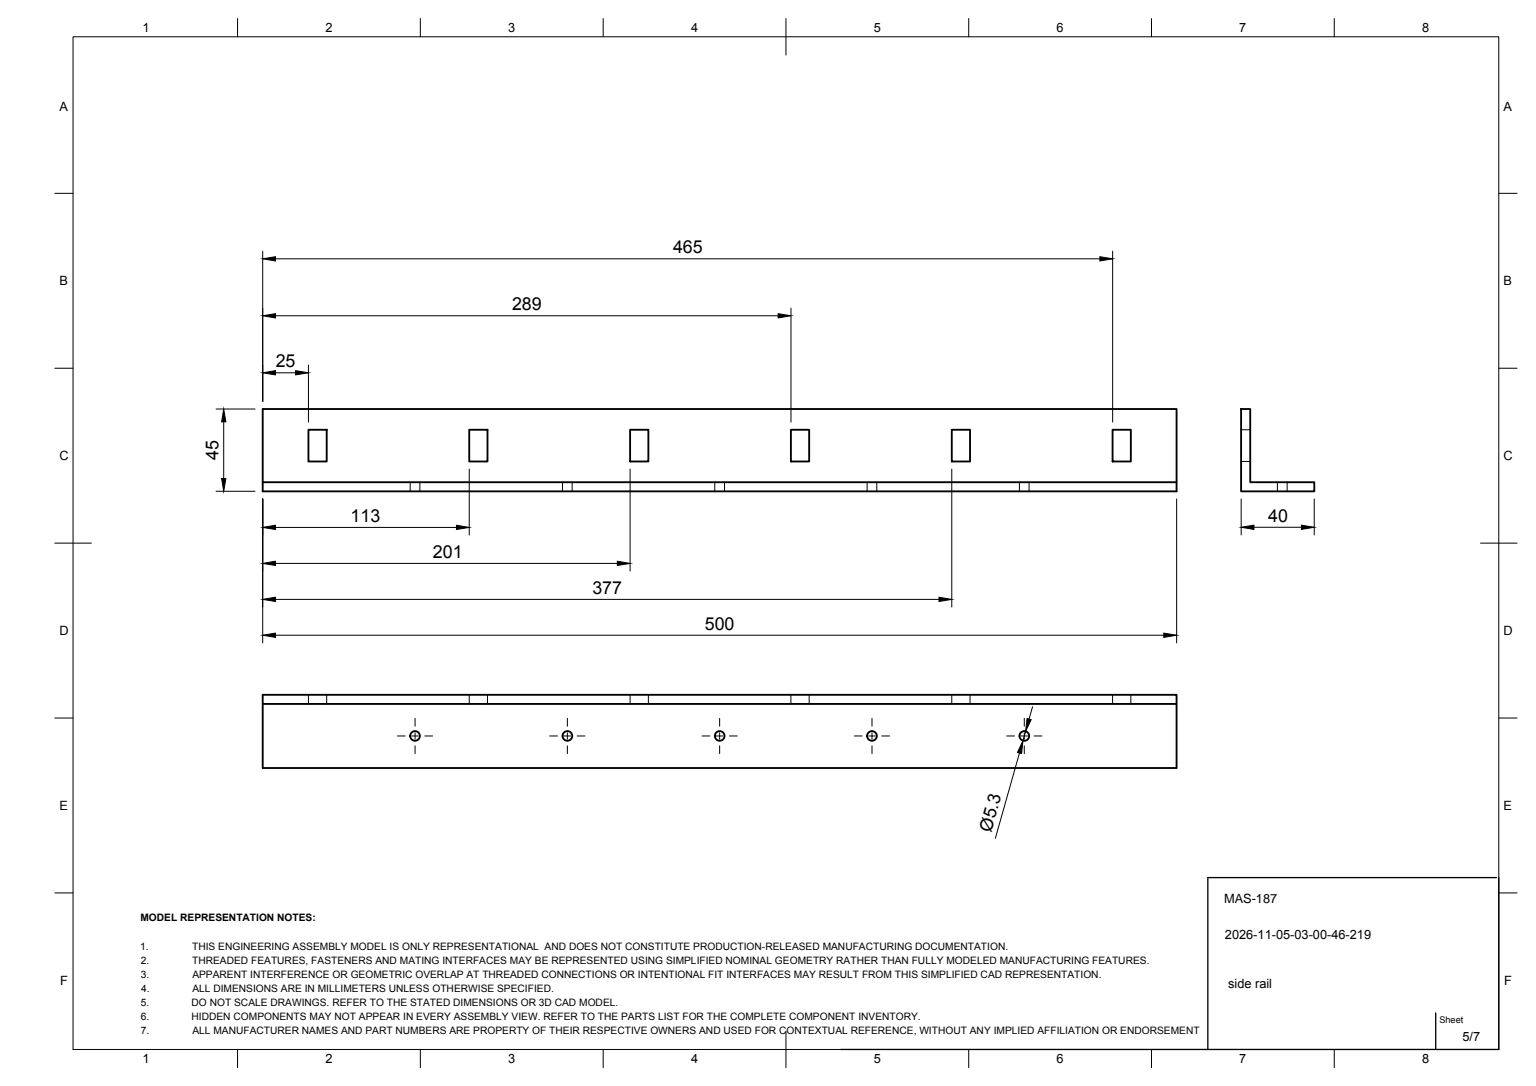
ISO-10303-21;
HEADER;
/* Generated by software containing ST-Developer
 * from STEP Tools, Inc. (www.steptools.com) 
 */

FILE_DESCRIPTION(
/* description */ ('STEP AP214'),
/* implementation_level */ '2;1');

FILE_NAME(
/* name */ 'side rail.step',
/* time_stamp */ '2026-11-04T19:00:26-08:00',
/* author */ (''),
/* organization */ (''),
/* preprocessor_version */ 'ST-DEVELOPER v20.2',
/* originating_system */ 'Autodesk Translation Framework v15.17.0.0',
/* authorisation */ '');

FILE_SCHEMA (('AUTOMOTIVE_DESIGN { 1 0 10303 214 3 1 1 }'));
ENDSEC;

DATA;
#10=MECHANICAL_DESIGN_GEOMETRIC_PRESENTATION_REPRESENTATION('',(#272),#5689);
#258=SHAPE_REPRESENTATION_RELATIONSHIP('SRR','None',#5759,#265);
#265=ADVANCED_BREP_SHAPE_REPRESENTATION('',(#279),#5683);
#272=STYLED_ITEM('',(#5803),#279);
#279=MANIFOLD_SOLID_BREP('Body1',#2962);
#309=FACE_BOUND('',#682,.T.);
#310=FACE_BOUND('',#683,.T.);
#311=FACE_BOUND('',#684,.T.);
#312=FACE_BOUND('',#685,.T.);
#313=FACE_BOUND('',#686,.T.);
#314=FACE_BOUND('',#687,.T.);
#315=FACE_BOUND('',#689,.T.);
#316=FACE_BOUND('',#690,.T.);
#317=FACE_BOUND('',#691,.T.);
#318=FACE_BOUND('',#692,.T.);
#319=FACE_BOUND('',#693,.T.);
#320=FACE_BOUND('',#694,.T.);
#321=FACE_BOUND('',#697,.T.);
#322=FACE_BOUND('',#698,.T.);
#323=FACE_BOUND('',#699,.T.);
#324=FACE_BOUND('',#700,.T.);
#325=FACE_BOUND('',#701,.T.);
#326=FACE_BOUND('',#703,.T.);
#327=FACE_BOUND('',#704,.T.);
#328=FACE_BOUND('',#705,.T.);
#329=FACE_BOUND('',#706,.T.);
#330=FACE_BOUND('',#707,.T.);
#361=PLANE('',#3124);
#362=PLANE('',#3125);
#363=PLANE('',#3126);
#364=PLANE('',#3127);
#365=PLANE('',#3128);
#366=PLANE('',#3129);
#367=PLANE('',#3130);
#368=PLANE('',#3131);
#369=PLANE('',#3132);
#370=PLANE('',#3133);
#371=PLANE('',#3134);
#372=PLANE('',#3135);
#373=PLANE('',#3136);
#374=PLANE('',#3137);
#375=PLANE('',#3138);
#376=PLANE('',#3139);
#377=PLANE('',#3140);
#378=PLANE('',#3141);
#379=PLANE('',#3142);
#380=PLANE('',#3143);
#381=PLANE('',#3144);
#382=PLANE('',#3145);
#383=PLANE('',#3146);
#384=PLANE('',#3147);
#385=PLANE('',#3148);
#386=PLANE('',#3149);
#387=PLANE('',#3150);
#388=PLANE('',#3151);
#389=PLANE('',#3152);
#390=PLANE('',#3153);
#391=PLANE('',#3154);
#392=PLANE('',#3155);
#474=FACE_OUTER_BOUND('',#657,.T.);
#475=FACE_OUTER_BOUND('',#658,.T.);
#476=FACE_OUTER_BOUND('',#659,.T.);
#477=FACE_OUTER_BOUND('',#660,.T.);
#478=FACE_OUTER_BOUND('',#661,.T.);
#479=FACE_OUTER_BOUND('',#662,.T.);
#480=FACE_OUTER_BOUND('',#663,.T.);
#481=FACE_OUTER_BOUND('',#664,.T.);
#482=FACE_OUTER_BOUND('',#665,.T.);
#483=FACE_OUTER_BOUND('',#666,.T.);
#484=FACE_OUTER_BOUND('',#667,.T.);
#485=FACE_OUTER_BOUND('',#668,.T.);
#486=FACE_OUTER_BOUND('',#669,.T.);
#487=FACE_OUTER_BOUND('',#670,.T.);
#488=FACE_OUTER_BOUND('',#671,.T.);
#489=FACE_OUTER_BOUND('',#672,.T.);
#490=FACE_OUTER_BOUND('',#673,.T.);
#491=FACE_OUTER_BOUND('',#674,.T.);
#492=FACE_OUTER_BOUND('',#675,.T.);
#493=FACE_OUTER_BOUND('',#676,.T.);
#494=FACE_OUTER_BOUND('',#677,.T.);
#495=FACE_OUTER_BOUND('',#678,.T.);
#496=FACE_OUTER_BOUND('',#679,.T.);
#497=FACE_OUTER_BOUND('',#680,.T.);
#498=FACE_OUTER_BOUND('',#681,.T.);
#499=FACE_OUTER_BOUND('',#688,.T.);
#500=FACE_OUTER_BOUND('',#695,.T.);
#501=FACE_OUTER_BOUND('',#696,.T.);
#502=FACE_OUTER_BOUND('',#702,.T.);
#503=FACE_OUTER_BOUND('',#708,.T.);
#504=FACE_OUTER_BOUND('',#709,.T.);
#505=FACE_OUTER_BOUND('',#710,.T.);
#506=FACE_OUTER_BOUND('',#711,.T.);
#507=FACE_OUTER_BOUND('',#712,.T.);
#508=FACE_OUTER_BOUND('',#713,.T.);
#509=FACE_OUTER_BOUND('',#714,.T.);
#510=FACE_OUTER_BOUND('',#715,.T.);
#657=EDGE_LOOP('',(#2192,#2193,#2194,#2195));
#658=EDGE_LOOP('',(#2196,#2197,#2198,#2199));
#659=EDGE_LOOP('',(#2200,#2201,#2202,#2203));
#660=EDGE_LOOP('',(#2204,#2205,#2206,#2207));
#661=EDGE_LOOP('',(#2208,#2209,#2210,#2211));
#662=EDGE_LOOP('',(#2212,#2213,#2214,#2215));
#663=EDGE_LOOP('',(#2216,#2217,#2218,#2219));
#664=EDGE_LOOP('',(#2220,#2221,#2222,#2223));
#665=EDGE_LOOP('',(#2224,#2225,#2226,#2227));
#666=EDGE_LOOP('',(#2228,#2229,#2230,#2231));
#667=EDGE_LOOP('',(#2232,#2233,#2234,#2235));
#668=EDGE_LOOP('',(#2236,#2237,#2238,#2239));
#669=EDGE_LOOP('',(#2240,#2241,#2242,#2243));
#670=EDGE_LOOP('',(#2244,#2245,#2246,#2247));
#671=EDGE_LOOP('',(#2248,#2249,#2250,#2251));
#672=EDGE_LOOP('',(#2252,#2253,#2254,#2255));
#673=EDGE_LOOP('',(#2256,#2257,#2258,#2259));
#674=EDGE_LOOP('',(#2260,#2261,#2262,#2263));
#675=EDGE_LOOP('',(#2264,#2265,#2266,#2267));
#676=EDGE_LOOP('',(#2268,#2269,#2270,#2271));
#677=EDGE_LOOP('',(#2272,#2273,#2274,#2275));
#678=EDGE_LOOP('',(#2276,#2277,#2278,#2279,#2280,#2281));
#679=EDGE_LOOP('',(#2282,#2283,#2284,#2285,#2286,#2287));
#680=EDGE_LOOP('',(#2288,#2289,#2290,#2291));
#681=EDGE_LOOP('',(#2292,#2293,#2294,#2295));
#682=EDGE_LOOP('',(#2296,#2297,#2298,#2299));
#683=EDGE_LOOP('',(#2300,#2301,#2302,#2303));
#684=EDGE_LOOP('',(#2304,#2305,#2306,#2307));
#685=EDGE_LOOP('',(#2308,#2309,#2310,#2311));
#686=EDGE_LOOP('',(#2312,#2313,#2314,#2315));
#687=EDGE_LOOP('',(#2316,#2317,#2318,#2319));
#688=EDGE_LOOP('',(#2320,#2321,#2322,#2323));
#689=EDGE_LOOP('',(#2324,#2325,#2326,#2327));
#690=EDGE_LOOP('',(#2328,#2329,#2330,#2331));
#691=EDGE_LOOP('',(#2332,#2333,#2334,#2335));
#692=EDGE_LOOP('',(#2336,#2337,#2338,#2339));
#693=EDGE_LOOP('',(#2340,#2341,#2342,#2343));
#694=EDGE_LOOP('',(#2344,#2345,#2346,#2347));
#695=EDGE_LOOP('',(#2348,#2349,#2350,#2351));
#696=EDGE_LOOP('',(#2352,#2353,#2354,#2355));
#697=EDGE_LOOP('',(#2356));
#698=EDGE_LOOP('',(#2357));
#699=EDGE_LOOP('',(#2358));
#700=EDGE_LOOP('',(#2359));
#701=EDGE_LOOP('',(#2360));
#702=EDGE_LOOP('',(#2361,#2362,#2363,#2364));
#703=EDGE_LOOP('',(#2365));
#704=EDGE_LOOP('',(#2366));
#705=EDGE_LOOP('',(#2367));
#706=EDGE_LOOP('',(#2368));
#707=EDGE_LOOP('',(#2369));
#708=EDGE_LOOP('',(#2370,#2371,#2372,#2373));
#709=EDGE_LOOP('',(#2374,#2375,#2376,#2377));
#710=EDGE_LOOP('',(#2378,#2379,#2380,#2381));
#711=EDGE_LOOP('',(#2382,#2383,#2384,#2385));
#712=EDGE_LOOP('',(#2386,#2387,#2388,#2389));
#713=EDGE_LOOP('',(#2390,#2391,#2392,#2393));
#714=EDGE_LOOP('',(#2394,#2395,#2396,#2397));
#715=EDGE_LOOP('',(#2398,#2399,#2400,#2401));
#880=LINE('',#4435,#1111);
#881=LINE('',#4441,#1112);
#882=LINE('',#4447,#1113);
#883=LINE('',#4453,#1114);
#884=LINE('',#4459,#1115);
#885=LINE('',#4464,#1116);
#886=LINE('',#4466,#1117);
#887=LINE('',#4468,#1118);
#888=LINE('',#4469,#1119);
#889=LINE('',#4472,#1120);
#890=LINE('',#4474,#1121);
#891=LINE('',#4475,#1122);
#892=LINE('',#4478,#1123);
#893=LINE('',#4480,#1124);
#894=LINE('',#4481,#1125);
#895=LINE('',#4483,#1126);
#896=LINE('',#4484,#1127);
#897=LINE('',#4488,#1128);
#898=LINE('',#4490,#1129);
#899=LINE('',#4492,#1130);
#900=LINE('',#4493,#1131);
#901=LINE('',#4496,#1132);
#902=LINE('',#4498,#1133);
#903=LINE('',#4499,#1134);
#904=LINE('',#4502,#1135);
#905=LINE('',#4504,#1136);
#906=LINE('',#4505,#1137);
#907=LINE('',#4507,#1138);
#908=LINE('',#4508,#1139);
#909=LINE('',#4512,#1140);
#910=LINE('',#4514,#1141);
#911=LINE('',#4516,#1142);
#912=LINE('',#4517,#1143);
#913=LINE('',#4520,#1144);
#914=LINE('',#4522,#1145);
#915=LINE('',#4523,#1146);
#916=LINE('',#4526,#1147);
#917=LINE('',#4528,#1148);
#918=LINE('',#4529,#1149);
#919=LINE('',#4531,#1150);
#920=LINE('',#4532,#1151);
#921=LINE('',#4536,#1152);
#922=LINE('',#4538,#1153);
#923=LINE('',#4540,#1154);
#924=LINE('',#4541,#1155);
#925=LINE('',#4544,#1156);
#926=LINE('',#4546,#1157);
#927=LINE('',#4547,#1158);
#928=LINE('',#4550,#1159);
#929=LINE('',#4552,#1160);
#930=LINE('',#4553,#1161);
#931=LINE('',#4555,#1162);
#932=LINE('',#4556,#1163);
#933=LINE('',#4560,#1164);
#934=LINE('',#4562,#1165);
#935=LINE('',#4564,#1166);
#936=LINE('',#4566,#1167);
#937=LINE('',#4568,#1168);
#938=LINE('',#4569,#1169);
#939=LINE('',#4573,#1170);
#940=LINE('',#4575,#1171);
#941=LINE('',#4577,#1172);
#942=LINE('',#4579,#1173);
#943=LINE('',#4581,#1174);
#944=LINE('',#4582,#1175);
#945=LINE('',#4584,#1176);
#946=LINE('',#4585,#1177);
#947=LINE('',#4587,#1178);
#948=LINE('',#4590,#1179);
#949=LINE('',#4592,#1180);
#950=LINE('',#4594,#1181);
#951=LINE('',#4595,#1182);
#952=LINE('',#4598,#1183);
#953=LINE('',#4600,#1184);
#954=LINE('',#4602,#1185);
#955=LINE('',#4603,#1186);
#956=LINE('',#4605,#1187);
#957=LINE('',#4608,#1188);
#958=LINE('',#4610,#1189);
#959=LINE('',#4612,#1190);
#960=LINE('',#4613,#1191);
#961=LINE('',#4616,#1192);
#962=LINE('',#4618,#1193);
#963=LINE('',#4620,#1194);
#964=LINE('',#4621,#1195);
#965=LINE('',#4623,#1196);
#966=LINE('',#4624,#1197);
#967=LINE('',#4628,#1198);
#968=LINE('',#4629,#1199);
#969=LINE('',#4631,#1200);
#970=LINE('',#4633,#1201);
#971=LINE('',#4636,#1202);
#972=LINE('',#4637,#1203);
#973=LINE('',#4639,#1204);
#974=LINE('',#4641,#1205);
#1111=VECTOR('',#3561,2.64999999999999);
#1112=VECTOR('',#3568,2.64999999999999);
#1113=VECTOR('',#3575,2.64999999999999);
#1114=VECTOR('',#3582,2.64999999999999);
#1115=VECTOR('',#3589,2.64999999999999);
#1116=VECTOR('',#3594,1000.);
#1117=VECTOR('',#3595,1000.);
#1118=VECTOR('',#3596,1000.);
#1119=VECTOR('',#3597,1000.);
#1120=VECTOR('',#3600,1000.);
#1121=VECTOR('',#3601,1000.);
#1122=VECTOR('',#3602,1000.);
#1123=VECTOR('',#3605,1000.);
#1124=VECTOR('',#3606,1000.);
#1125=VECTOR('',#3607,1000.);
#1126=VECTOR('',#3610,1000.);
#1127=VECTOR('',#3611,1000.);
#1128=VECTOR('',#3614,1000.);
#1129=VECTOR('',#3615,1000.);
#1130=VECTOR('',#3616,1000.);
#1131=VECTOR('',#3617,1000.);
#1132=VECTOR('',#3620,1000.);
#1133=VECTOR('',#3621,1000.);
#1134=VECTOR('',#3622,1000.);
#1135=VECTOR('',#3625,1000.);
#1136=VECTOR('',#3626,1000.);
#1137=VECTOR('',#3627,1000.);
#1138=VECTOR('',#3630,1000.);
#1139=VECTOR('',#3631,1000.);
#1140=VECTOR('',#3634,1000.);
#1141=VECTOR('',#3635,1000.);
#1142=VECTOR('',#3636,1000.);
#1143=VECTOR('',#3637,1000.);
#1144=VECTOR('',#3640,1000.);
#1145=VECTOR('',#3641,1000.);
#1146=VECTOR('',#3642,1000.);
#1147=VECTOR('',#3645,1000.);
#1148=VECTOR('',#3646,1000.);
#1149=VECTOR('',#3647,1000.);
#1150=VECTOR('',#3650,1000.);
#1151=VECTOR('',#3651,1000.);
#1152=VECTOR('',#3654,1000.);
#1153=VECTOR('',#3655,1000.);
#1154=VECTOR('',#3656,1000.);
#1155=VECTOR('',#3657,1000.);
#1156=VECTOR('',#3660,1000.);
#1157=VECTOR('',#3661,1000.);
#1158=VECTOR('',#3662,1000.);
#1159=VECTOR('',#3665,1000.);
#1160=VECTOR('',#3666,1000.);
#1161=VECTOR('',#3667,1000.);
#1162=VECTOR('',#3670,1000.);
#1163=VECTOR('',#3671,1000.);
#1164=VECTOR('',#3674,1000.);
#1165=VECTOR('',#3675,1000.);
#1166=VECTOR('',#3676,1000.);
#1167=VECTOR('',#3677,1000.);
#1168=VECTOR('',#3678,1000.);
#1169=VECTOR('',#3679,1000.);
#1170=VECTOR('',#3682,1000.);
#1171=VECTOR('',#3683,1000.);
#1172=VECTOR('',#3684,1000.);
#1173=VECTOR('',#3685,1000.);
#1174=VECTOR('',#3686,1000.);
#1175=VECTOR('',#3687,1000.);
#1176=VECTOR('',#3690,1000.);
#1177=VECTOR('',#3691,1000.);
#1178=VECTOR('',#3694,1000.);
#1179=VECTOR('',#3695,1000.);
#1180=VECTOR('',#3696,1000.);
#1181=VECTOR('',#3697,1000.);
#1182=VECTOR('',#3698,1000.);
#1183=VECTOR('',#3699,1000.);
#1184=VECTOR('',#3700,1000.);
#1185=VECTOR('',#3701,1000.);
#1186=VECTOR('',#3702,1000.);
#1187=VECTOR('',#3705,1000.);
#1188=VECTOR('',#3706,1000.);
#1189=VECTOR('',#3707,1000.);
#1190=VECTOR('',#3708,1000.);
#1191=VECTOR('',#3709,1000.);
#1192=VECTOR('',#3710,1000.);
#1193=VECTOR('',#3711,1000.);
#1194=VECTOR('',#3712,1000.);
#1195=VECTOR('',#3713,1000.);
#1196=VECTOR('',#3716,1000.);
#1197=VECTOR('',#3717,1000.);
#1198=VECTOR('',#3724,1000.);
#1199=VECTOR('',#3725,1000.);
#1200=VECTOR('',#3728,1000.);
#1201=VECTOR('',#3731,1000.);
#1202=VECTOR('',#3736,1000.);
#1203=VECTOR('',#3737,1000.);
#1204=VECTOR('',#3740,1000.);
#1205=VECTOR('',#3743,1000.);
#1308=CIRCLE('',#3110,2.64999999999999);
#1309=CIRCLE('',#3111,2.64999999999999);
#1310=CIRCLE('',#3113,2.64999999999999);
#1311=CIRCLE('',#3114,2.64999999999999);
#1312=CIRCLE('',#3116,2.64999999999999);
#1313=CIRCLE('',#3117,2.64999999999999);
#1314=CIRCLE('',#3119,2.64999999999999);
#1315=CIRCLE('',#3120,2.64999999999999);
#1316=CIRCLE('',#3122,2.64999999999999);
#1317=CIRCLE('',#3123,2.64999999999999);
#1455=VERTEX_POINT('',#4432);
#1456=VERTEX_POINT('',#4434);
#1457=VERTEX_POINT('',#4438);
#1458=VERTEX_POINT('',#4440);
#1459=VERTEX_POINT('',#4444);
#1460=VERTEX_POINT('',#4446);
#1461=VERTEX_POINT('',#4450);
#1462=VERTEX_POINT('',#4452);
#1463=VERTEX_POINT('',#4456);
#1464=VERTEX_POINT('',#4458);
#1465=VERTEX_POINT('',#4462);
#1466=VERTEX_POINT('',#4463);
#1467=VERTEX_POINT('',#4465);
#1468=VERTEX_POINT('',#4467);
#1469=VERTEX_POINT('',#4471);
#1470=VERTEX_POINT('',#4473);
#1471=VERTEX_POINT('',#4477);
#1472=VERTEX_POINT('',#4479);
#1473=VERTEX_POINT('',#4486);
#1474=VERTEX_POINT('',#4487);
#1475=VERTEX_POINT('',#4489);
#1476=VERTEX_POINT('',#4491);
#1477=VERTEX_POINT('',#4495);
#1478=VERTEX_POINT('',#4497);
#1479=VERTEX_POINT('',#4501);
#1480=VERTEX_POINT('',#4503);
#1481=VERTEX_POINT('',#4510);
#1482=VERTEX_POINT('',#4511);
#1483=VERTEX_POINT('',#4513);
#1484=VERTEX_POINT('',#4515);
#1485=VERTEX_POINT('',#4519);
#1486=VERTEX_POINT('',#4521);
#1487=VERTEX_POINT('',#4525);
#1488=VERTEX_POINT('',#4527);
#1489=VERTEX_POINT('',#4534);
#1490=VERTEX_POINT('',#4535);
#1491=VERTEX_POINT('',#4537);
#1492=VERTEX_POINT('',#4539);
#1493=VERTEX_POINT('',#4543);
#1494=VERTEX_POINT('',#4545);
#1495=VERTEX_POINT('',#4549);
#1496=VERTEX_POINT('',#4551);
#1497=VERTEX_POINT('',#4558);
#1498=VERTEX_POINT('',#4559);
#1499=VERTEX_POINT('',#4561);
#1500=VERTEX_POINT('',#4563);
#1501=VERTEX_POINT('',#4565);
#1502=VERTEX_POINT('',#4567);
#1503=VERTEX_POINT('',#4571);
#1504=VERTEX_POINT('',#4572);
#1505=VERTEX_POINT('',#4574);
#1506=VERTEX_POINT('',#4576);
#1507=VERTEX_POINT('',#4578);
#1508=VERTEX_POINT('',#4580);
#1509=VERTEX_POINT('',#4588);
#1510=VERTEX_POINT('',#4589);
#1511=VERTEX_POINT('',#4591);
#1512=VERTEX_POINT('',#4593);
#1513=VERTEX_POINT('',#4596);
#1514=VERTEX_POINT('',#4597);
#1515=VERTEX_POINT('',#4599);
#1516=VERTEX_POINT('',#4601);
#1517=VERTEX_POINT('',#4606);
#1518=VERTEX_POINT('',#4607);
#1519=VERTEX_POINT('',#4609);
#1520=VERTEX_POINT('',#4611);
#1521=VERTEX_POINT('',#4614);
#1522=VERTEX_POINT('',#4615);
#1523=VERTEX_POINT('',#4617);
#1524=VERTEX_POINT('',#4619);
#1724=EDGE_CURVE('',#1455,#1455,#1308,.T.);
#1725=EDGE_CURVE('',#1455,#1456,#880,.T.);
#1726=EDGE_CURVE('',#1456,#1456,#1309,.T.);
#1727=EDGE_CURVE('',#1457,#1457,#1310,.T.);
#1728=EDGE_CURVE('',#1457,#1458,#881,.T.);
#1729=EDGE_CURVE('',#1458,#1458,#1311,.T.);
#1730=EDGE_CURVE('',#1459,#1459,#1312,.T.);
#1731=EDGE_CURVE('',#1459,#1460,#882,.T.);
#1732=EDGE_CURVE('',#1460,#1460,#1313,.T.);
#1733=EDGE_CURVE('',#1461,#1461,#1314,.T.);
#1734=EDGE_CURVE('',#1461,#1462,#883,.T.);
#1735=EDGE_CURVE('',#1462,#1462,#1315,.T.);
#1736=EDGE_CURVE('',#1463,#1463,#1316,.T.);
#1737=EDGE_CURVE('',#1463,#1464,#884,.T.);
#1738=EDGE_CURVE('',#1464,#1464,#1317,.T.);
#1739=EDGE_CURVE('',#1465,#1466,#885,.T.);
#1740=EDGE_CURVE('',#1466,#1467,#886,.T.);
#1741=EDGE_CURVE('',#1468,#1467,#887,.T.);
#1742=EDGE_CURVE('',#1465,#1468,#888,.T.);
#1743=EDGE_CURVE('',#1467,#1469,#889,.T.);
#1744=EDGE_CURVE('',#1470,#1469,#890,.T.);
#1745=EDGE_CURVE('',#1468,#1470,#891,.T.);
#1746=EDGE_CURVE('',#1469,#1471,#892,.T.);
#1747=EDGE_CURVE('',#1472,#1471,#893,.T.);
#1748=EDGE_CURVE('',#1470,#1472,#894,.T.);
#1749=EDGE_CURVE('',#1471,#1466,#895,.T.);
#1750=EDGE_CURVE('',#1472,#1465,#896,.T.);
#1751=EDGE_CURVE('',#1473,#1474,#897,.T.);
#1752=EDGE_CURVE('',#1474,#1475,#898,.T.);
#1753=EDGE_CURVE('',#1476,#1475,#899,.T.);
#1754=EDGE_CURVE('',#1473,#1476,#900,.T.);
#1755=EDGE_CURVE('',#1475,#1477,#901,.T.);
#1756=EDGE_CURVE('',#1478,#1477,#902,.T.);
#1757=EDGE_CURVE('',#1476,#1478,#903,.T.);
#1758=EDGE_CURVE('',#1477,#1479,#904,.T.);
#1759=EDGE_CURVE('',#1480,#1479,#905,.T.);
#1760=EDGE_CURVE('',#1478,#1480,#906,.T.);
#1761=EDGE_CURVE('',#1479,#1474,#907,.T.);
#1762=EDGE_CURVE('',#1480,#1473,#908,.T.);
#1763=EDGE_CURVE('',#1481,#1482,#909,.T.);
#1764=EDGE_CURVE('',#1482,#1483,#910,.T.);
#1765=EDGE_CURVE('',#1484,#1483,#911,.T.);
#1766=EDGE_CURVE('',#1481,#1484,#912,.T.);
#1767=EDGE_CURVE('',#1483,#1485,#913,.T.);
#1768=EDGE_CURVE('',#1486,#1485,#914,.T.);
#1769=EDGE_CURVE('',#1484,#1486,#915,.T.);
#1770=EDGE_CURVE('',#1485,#1487,#916,.T.);
#1771=EDGE_CURVE('',#1488,#1487,#917,.T.);
#1772=EDGE_CURVE('',#1486,#1488,#918,.T.);
#1773=EDGE_CURVE('',#1487,#1482,#919,.T.);
#1774=EDGE_CURVE('',#1488,#1481,#920,.T.);
#1775=EDGE_CURVE('',#1489,#1490,#921,.T.);
#1776=EDGE_CURVE('',#1490,#1491,#922,.T.);
#1777=EDGE_CURVE('',#1492,#1491,#923,.T.);
#1778=EDGE_CURVE('',#1489,#1492,#924,.T.);
#1779=EDGE_CURVE('',#1491,#1493,#925,.T.);
#1780=EDGE_CURVE('',#1494,#1493,#926,.T.);
#1781=EDGE_CURVE('',#1492,#1494,#927,.T.);
#1782=EDGE_CURVE('',#1493,#1495,#928,.T.);
#1783=EDGE_CURVE('',#1496,#1495,#929,.T.);
#1784=EDGE_CURVE('',#1494,#1496,#930,.T.);
#1785=EDGE_CURVE('',#1495,#1490,#931,.T.);
#1786=EDGE_CURVE('',#1496,#1489,#932,.T.);
#1787=EDGE_CURVE('',#1497,#1498,#933,.T.);
#1788=EDGE_CURVE('',#1498,#1499,#934,.T.);
#1789=EDGE_CURVE('',#1499,#1500,#935,.T.);
#1790=EDGE_CURVE('',#1501,#1500,#936,.T.);
#1791=EDGE_CURVE('',#1502,#1501,#937,.T.);
#1792=EDGE_CURVE('',#1502,#1497,#938,.T.);
#1793=EDGE_CURVE('',#1503,#1504,#939,.T.);
#1794=EDGE_CURVE('',#1505,#1504,#940,.T.);
#1795=EDGE_CURVE('',#1506,#1505,#941,.T.);
#1796=EDGE_CURVE('',#1507,#1506,#942,.T.);
#1797=EDGE_CURVE('',#1508,#1507,#943,.T.);
#1798=EDGE_CURVE('',#1508,#1503,#944,.T.);
#1799=EDGE_CURVE('',#1504,#1497,#945,.T.);
#1800=EDGE_CURVE('',#1505,#1502,#946,.T.);
#1801=EDGE_CURVE('',#1506,#1501,#947,.T.);
#1802=EDGE_CURVE('',#1509,#1510,#948,.T.);
#1803=EDGE_CURVE('',#1511,#1509,#949,.T.);
#1804=EDGE_CURVE('',#1512,#1511,#950,.T.);
#1805=EDGE_CURVE('',#1510,#1512,#951,.T.);
#1806=EDGE_CURVE('',#1513,#1514,#952,.T.);
#1807=EDGE_CURVE('',#1515,#1513,#953,.T.);
#1808=EDGE_CURVE('',#1516,#1515,#954,.T.);
#1809=EDGE_CURVE('',#1514,#1516,#955,.T.);
#1810=EDGE_CURVE('',#1498,#1503,#956,.T.);
#1811=EDGE_CURVE('',#1517,#1518,#957,.T.);
#1812=EDGE_CURVE('',#1518,#1519,#958,.T.);
#1813=EDGE_CURVE('',#1519,#1520,#959,.T.);
#1814=EDGE_CURVE('',#1520,#1517,#960,.T.);
#1815=EDGE_CURVE('',#1521,#1522,#961,.T.);
#1816=EDGE_CURVE('',#1522,#1523,#962,.T.);
#1817=EDGE_CURVE('',#1523,#1524,#963,.T.);
#1818=EDGE_CURVE('',#1524,#1521,#964,.T.);
#1819=EDGE_CURVE('',#1500,#1507,#965,.T.);
#1820=EDGE_CURVE('',#1499,#1508,#966,.T.);
#1821=EDGE_CURVE('',#1521,#1515,#967,.T.);
#1822=EDGE_CURVE('',#1522,#1513,#968,.T.);
#1823=EDGE_CURVE('',#1524,#1516,#969,.T.);
#1824=EDGE_CURVE('',#1523,#1514,#970,.T.);
#1825=EDGE_CURVE('',#1517,#1511,#971,.T.);
#1826=EDGE_CURVE('',#1518,#1509,#972,.T.);
#1827=EDGE_CURVE('',#1520,#1512,#973,.T.);
#1828=EDGE_CURVE('',#1519,#1510,#974,.T.);
#2192=ORIENTED_EDGE('',*,*,#1724,.F.);
#2193=ORIENTED_EDGE('',*,*,#1725,.T.);
#2194=ORIENTED_EDGE('',*,*,#1726,.T.);
#2195=ORIENTED_EDGE('',*,*,#1725,.F.);
#2196=ORIENTED_EDGE('',*,*,#1727,.F.);
#2197=ORIENTED_EDGE('',*,*,#1728,.T.);
#2198=ORIENTED_EDGE('',*,*,#1729,.T.);
#2199=ORIENTED_EDGE('',*,*,#1728,.F.);
#2200=ORIENTED_EDGE('',*,*,#1730,.F.);
#2201=ORIENTED_EDGE('',*,*,#1731,.T.);
#2202=ORIENTED_EDGE('',*,*,#1732,.T.);
#2203=ORIENTED_EDGE('',*,*,#1731,.F.);
#2204=ORIENTED_EDGE('',*,*,#1733,.F.);
#2205=ORIENTED_EDGE('',*,*,#1734,.T.);
#2206=ORIENTED_EDGE('',*,*,#1735,.T.);
#2207=ORIENTED_EDGE('',*,*,#1734,.F.);
#2208=ORIENTED_EDGE('',*,*,#1736,.F.);
#2209=ORIENTED_EDGE('',*,*,#1737,.T.);
#2210=ORIENTED_EDGE('',*,*,#1738,.T.);
#2211=ORIENTED_EDGE('',*,*,#1737,.F.);
#2212=ORIENTED_EDGE('',*,*,#1739,.T.);
#2213=ORIENTED_EDGE('',*,*,#1740,.T.);
#2214=ORIENTED_EDGE('',*,*,#1741,.F.);
#2215=ORIENTED_EDGE('',*,*,#1742,.F.);
#2216=ORIENTED_EDGE('',*,*,#1741,.T.);
#2217=ORIENTED_EDGE('',*,*,#1743,.T.);
#2218=ORIENTED_EDGE('',*,*,#1744,.F.);
#2219=ORIENTED_EDGE('',*,*,#1745,.F.);
#2220=ORIENTED_EDGE('',*,*,#1744,.T.);
#2221=ORIENTED_EDGE('',*,*,#1746,.T.);
#2222=ORIENTED_EDGE('',*,*,#1747,.F.);
#2223=ORIENTED_EDGE('',*,*,#1748,.F.);
#2224=ORIENTED_EDGE('',*,*,#1747,.T.);
#2225=ORIENTED_EDGE('',*,*,#1749,.T.);
#2226=ORIENTED_EDGE('',*,*,#1739,.F.);
#2227=ORIENTED_EDGE('',*,*,#1750,.F.);
#2228=ORIENTED_EDGE('',*,*,#1751,.T.);
#2229=ORIENTED_EDGE('',*,*,#1752,.T.);
#2230=ORIENTED_EDGE('',*,*,#1753,.F.);
#2231=ORIENTED_EDGE('',*,*,#1754,.F.);
#2232=ORIENTED_EDGE('',*,*,#1753,.T.);
#2233=ORIENTED_EDGE('',*,*,#1755,.T.);
#2234=ORIENTED_EDGE('',*,*,#1756,.F.);
#2235=ORIENTED_EDGE('',*,*,#1757,.F.);
#2236=ORIENTED_EDGE('',*,*,#1756,.T.);
#2237=ORIENTED_EDGE('',*,*,#1758,.T.);
#2238=ORIENTED_EDGE('',*,*,#1759,.F.);
#2239=ORIENTED_EDGE('',*,*,#1760,.F.);
#2240=ORIENTED_EDGE('',*,*,#1759,.T.);
#2241=ORIENTED_EDGE('',*,*,#1761,.T.);
#2242=ORIENTED_EDGE('',*,*,#1751,.F.);
#2243=ORIENTED_EDGE('',*,*,#1762,.F.);
#2244=ORIENTED_EDGE('',*,*,#1763,.T.);
#2245=ORIENTED_EDGE('',*,*,#1764,.T.);
#2246=ORIENTED_EDGE('',*,*,#1765,.F.);
#2247=ORIENTED_EDGE('',*,*,#1766,.F.);
#2248=ORIENTED_EDGE('',*,*,#1765,.T.);
#2249=ORIENTED_EDGE('',*,*,#1767,.T.);
#2250=ORIENTED_EDGE('',*,*,#1768,.F.);
#2251=ORIENTED_EDGE('',*,*,#1769,.F.);
#2252=ORIENTED_EDGE('',*,*,#1768,.T.);
#2253=ORIENTED_EDGE('',*,*,#1770,.T.);
#2254=ORIENTED_EDGE('',*,*,#1771,.F.);
#2255=ORIENTED_EDGE('',*,*,#1772,.F.);
#2256=ORIENTED_EDGE('',*,*,#1771,.T.);
#2257=ORIENTED_EDGE('',*,*,#1773,.T.);
#2258=ORIENTED_EDGE('',*,*,#1763,.F.);
#2259=ORIENTED_EDGE('',*,*,#1774,.F.);
#2260=ORIENTED_EDGE('',*,*,#1775,.T.);
#2261=ORIENTED_EDGE('',*,*,#1776,.T.);
#2262=ORIENTED_EDGE('',*,*,#1777,.F.);
#2263=ORIENTED_EDGE('',*,*,#1778,.F.);
#2264=ORIENTED_EDGE('',*,*,#1777,.T.);
#2265=ORIENTED_EDGE('',*,*,#1779,.T.);
#2266=ORIENTED_EDGE('',*,*,#1780,.F.);
#2267=ORIENTED_EDGE('',*,*,#1781,.F.);
#2268=ORIENTED_EDGE('',*,*,#1780,.T.);
#2269=ORIENTED_EDGE('',*,*,#1782,.T.);
#2270=ORIENTED_EDGE('',*,*,#1783,.F.);
#2271=ORIENTED_EDGE('',*,*,#1784,.F.);
#2272=ORIENTED_EDGE('',*,*,#1783,.T.);
#2273=ORIENTED_EDGE('',*,*,#1785,.T.);
#2274=ORIENTED_EDGE('',*,*,#1775,.F.);
#2275=ORIENTED_EDGE('',*,*,#1786,.F.);
#2276=ORIENTED_EDGE('',*,*,#1787,.T.);
#2277=ORIENTED_EDGE('',*,*,#1788,.T.);
#2278=ORIENTED_EDGE('',*,*,#1789,.T.);
#2279=ORIENTED_EDGE('',*,*,#1790,.F.);
#2280=ORIENTED_EDGE('',*,*,#1791,.F.);
#2281=ORIENTED_EDGE('',*,*,#1792,.T.);
#2282=ORIENTED_EDGE('',*,*,#1793,.T.);
#2283=ORIENTED_EDGE('',*,*,#1794,.F.);
#2284=ORIENTED_EDGE('',*,*,#1795,.F.);
#2285=ORIENTED_EDGE('',*,*,#1796,.F.);
#2286=ORIENTED_EDGE('',*,*,#1797,.F.);
#2287=ORIENTED_EDGE('',*,*,#1798,.T.);
#2288=ORIENTED_EDGE('',*,*,#1799,.T.);
#2289=ORIENTED_EDGE('',*,*,#1792,.F.);
#2290=ORIENTED_EDGE('',*,*,#1800,.F.);
#2291=ORIENTED_EDGE('',*,*,#1794,.T.);
#2292=ORIENTED_EDGE('',*,*,#1791,.T.);
#2293=ORIENTED_EDGE('',*,*,#1801,.F.);
#2294=ORIENTED_EDGE('',*,*,#1795,.T.);
#2295=ORIENTED_EDGE('',*,*,#1800,.T.);
#2296=ORIENTED_EDGE('',*,*,#1785,.F.);
#2297=ORIENTED_EDGE('',*,*,#1782,.F.);
#2298=ORIENTED_EDGE('',*,*,#1779,.F.);
#2299=ORIENTED_EDGE('',*,*,#1776,.F.);
#2300=ORIENTED_EDGE('',*,*,#1773,.F.);
#2301=ORIENTED_EDGE('',*,*,#1770,.F.);
#2302=ORIENTED_EDGE('',*,*,#1767,.F.);
#2303=ORIENTED_EDGE('',*,*,#1764,.F.);
#2304=ORIENTED_EDGE('',*,*,#1761,.F.);
#2305=ORIENTED_EDGE('',*,*,#1758,.F.);
#2306=ORIENTED_EDGE('',*,*,#1755,.F.);
#2307=ORIENTED_EDGE('',*,*,#1752,.F.);
#2308=ORIENTED_EDGE('',*,*,#1749,.F.);
#2309=ORIENTED_EDGE('',*,*,#1746,.F.);
#2310=ORIENTED_EDGE('',*,*,#1743,.F.);
#2311=ORIENTED_EDGE('',*,*,#1740,.F.);
#2312=ORIENTED_EDGE('',*,*,#1802,.F.);
#2313=ORIENTED_EDGE('',*,*,#1803,.F.);
#2314=ORIENTED_EDGE('',*,*,#1804,.F.);
#2315=ORIENTED_EDGE('',*,*,#1805,.F.);
#2316=ORIENTED_EDGE('',*,*,#1806,.F.);
#2317=ORIENTED_EDGE('',*,*,#1807,.F.);
#2318=ORIENTED_EDGE('',*,*,#1808,.F.);
#2319=ORIENTED_EDGE('',*,*,#1809,.F.);
#2320=ORIENTED_EDGE('',*,*,#1787,.F.);
#2321=ORIENTED_EDGE('',*,*,#1799,.F.);
#2322=ORIENTED_EDGE('',*,*,#1793,.F.);
#2323=ORIENTED_EDGE('',*,*,#1810,.F.);
#2324=ORIENTED_EDGE('',*,*,#1786,.T.);
#2325=ORIENTED_EDGE('',*,*,#1778,.T.);
#2326=ORIENTED_EDGE('',*,*,#1781,.T.);
#2327=ORIENTED_EDGE('',*,*,#1784,.T.);
#2328=ORIENTED_EDGE('',*,*,#1774,.T.);
#2329=ORIENTED_EDGE('',*,*,#1766,.T.);
#2330=ORIENTED_EDGE('',*,*,#1769,.T.);
#2331=ORIENTED_EDGE('',*,*,#1772,.T.);
#2332=ORIENTED_EDGE('',*,*,#1762,.T.);
#2333=ORIENTED_EDGE('',*,*,#1754,.T.);
#2334=ORIENTED_EDGE('',*,*,#1757,.T.);
#2335=ORIENTED_EDGE('',*,*,#1760,.T.);
#2336=ORIENTED_EDGE('',*,*,#1750,.T.);
#2337=ORIENTED_EDGE('',*,*,#1742,.T.);
#2338=ORIENTED_EDGE('',*,*,#1745,.T.);
#2339=ORIENTED_EDGE('',*,*,#1748,.T.);
#2340=ORIENTED_EDGE('',*,*,#1811,.T.);
#2341=ORIENTED_EDGE('',*,*,#1812,.T.);
#2342=ORIENTED_EDGE('',*,*,#1813,.T.);
#2343=ORIENTED_EDGE('',*,*,#1814,.T.);
#2344=ORIENTED_EDGE('',*,*,#1815,.T.);
#2345=ORIENTED_EDGE('',*,*,#1816,.T.);
#2346=ORIENTED_EDGE('',*,*,#1817,.T.);
#2347=ORIENTED_EDGE('',*,*,#1818,.T.);
#2348=ORIENTED_EDGE('',*,*,#1819,.F.);
#2349=ORIENTED_EDGE('',*,*,#1789,.F.);
#2350=ORIENTED_EDGE('',*,*,#1820,.T.);
#2351=ORIENTED_EDGE('',*,*,#1797,.T.);
#2352=ORIENTED_EDGE('',*,*,#1810,.T.);
#2353=ORIENTED_EDGE('',*,*,#1798,.F.);
#2354=ORIENTED_EDGE('',*,*,#1820,.F.);
#2355=ORIENTED_EDGE('',*,*,#1788,.F.);
#2356=ORIENTED_EDGE('',*,*,#1724,.T.);
#2357=ORIENTED_EDGE('',*,*,#1727,.T.);
#2358=ORIENTED_EDGE('',*,*,#1730,.T.);
#2359=ORIENTED_EDGE('',*,*,#1733,.T.);
#2360=ORIENTED_EDGE('',*,*,#1736,.T.);
#2361=ORIENTED_EDGE('',*,*,#1796,.T.);
#2362=ORIENTED_EDGE('',*,*,#1801,.T.);
#2363=ORIENTED_EDGE('',*,*,#1790,.T.);
#2364=ORIENTED_EDGE('',*,*,#1819,.T.);
#2365=ORIENTED_EDGE('',*,*,#1726,.F.);
#2366=ORIENTED_EDGE('',*,*,#1729,.F.);
#2367=ORIENTED_EDGE('',*,*,#1732,.F.);
#2368=ORIENTED_EDGE('',*,*,#1735,.F.);
#2369=ORIENTED_EDGE('',*,*,#1738,.F.);
#2370=ORIENTED_EDGE('',*,*,#1821,.T.);
#2371=ORIENTED_EDGE('',*,*,#1807,.T.);
#2372=ORIENTED_EDGE('',*,*,#1822,.F.);
#2373=ORIENTED_EDGE('',*,*,#1815,.F.);
#2374=ORIENTED_EDGE('',*,*,#1823,.T.);
#2375=ORIENTED_EDGE('',*,*,#1808,.T.);
#2376=ORIENTED_EDGE('',*,*,#1821,.F.);
#2377=ORIENTED_EDGE('',*,*,#1818,.F.);
#2378=ORIENTED_EDGE('',*,*,#1824,.T.);
#2379=ORIENTED_EDGE('',*,*,#1809,.T.);
#2380=ORIENTED_EDGE('',*,*,#1823,.F.);
#2381=ORIENTED_EDGE('',*,*,#1817,.F.);
#2382=ORIENTED_EDGE('',*,*,#1822,.T.);
#2383=ORIENTED_EDGE('',*,*,#1806,.T.);
#2384=ORIENTED_EDGE('',*,*,#1824,.F.);
#2385=ORIENTED_EDGE('',*,*,#1816,.F.);
#2386=ORIENTED_EDGE('',*,*,#1825,.T.);
#2387=ORIENTED_EDGE('',*,*,#1803,.T.);
#2388=ORIENTED_EDGE('',*,*,#1826,.F.);
#2389=ORIENTED_EDGE('',*,*,#1811,.F.);
#2390=ORIENTED_EDGE('',*,*,#1827,.T.);
#2391=ORIENTED_EDGE('',*,*,#1804,.T.);
#2392=ORIENTED_EDGE('',*,*,#1825,.F.);
#2393=ORIENTED_EDGE('',*,*,#1814,.F.);
#2394=ORIENTED_EDGE('',*,*,#1828,.T.);
#2395=ORIENTED_EDGE('',*,*,#1805,.T.);
#2396=ORIENTED_EDGE('',*,*,#1827,.F.);
#2397=ORIENTED_EDGE('',*,*,#1813,.F.);
#2398=ORIENTED_EDGE('',*,*,#1826,.T.);
#2399=ORIENTED_EDGE('',*,*,#1802,.T.);
#2400=ORIENTED_EDGE('',*,*,#1828,.F.);
#2401=ORIENTED_EDGE('',*,*,#1812,.F.);
#2782=CYLINDRICAL_SURFACE('',#3109,2.64999999999999);
#2783=CYLINDRICAL_SURFACE('',#3112,2.64999999999999);
#2784=CYLINDRICAL_SURFACE('',#3115,2.64999999999999);
#2785=CYLINDRICAL_SURFACE('',#3118,2.64999999999999);
#2786=CYLINDRICAL_SURFACE('',#3121,2.64999999999999);
#2834=ADVANCED_FACE('',(#474),#2782,.F.);
#2835=ADVANCED_FACE('',(#475),#2783,.F.);
#2836=ADVANCED_FACE('',(#476),#2784,.F.);
#2837=ADVANCED_FACE('',(#477),#2785,.F.);
#2838=ADVANCED_FACE('',(#478),#2786,.F.);
#2839=ADVANCED_FACE('',(#479),#361,.F.);
#2840=ADVANCED_FACE('',(#480),#362,.F.);
#2841=ADVANCED_FACE('',(#481),#363,.F.);
#2842=ADVANCED_FACE('',(#482),#364,.F.);
#2843=ADVANCED_FACE('',(#483),#365,.F.);
#2844=ADVANCED_FACE('',(#484),#366,.F.);
#2845=ADVANCED_FACE('',(#485),#367,.F.);
#2846=ADVANCED_FACE('',(#486),#368,.F.);
#2847=ADVANCED_FACE('',(#487),#369,.F.);
#2848=ADVANCED_FACE('',(#488),#370,.F.);
#2849=ADVANCED_FACE('',(#489),#371,.F.);
#2850=ADVANCED_FACE('',(#490),#372,.F.);
#2851=ADVANCED_FACE('',(#491),#373,.F.);
#2852=ADVANCED_FACE('',(#492),#374,.F.);
#2853=ADVANCED_FACE('',(#493),#375,.F.);
#2854=ADVANCED_FACE('',(#494),#376,.F.);
#2855=ADVANCED_FACE('',(#495),#377,.F.);
#2856=ADVANCED_FACE('',(#496),#378,.F.);
#2857=ADVANCED_FACE('',(#497),#379,.F.);
#2858=ADVANCED_FACE('',(#498,#309,#310,#311,#312,#313,#314),#380,.F.);
#2859=ADVANCED_FACE('',(#499,#315,#316,#317,#318,#319,#320),#381,.T.);
#2860=ADVANCED_FACE('',(#500),#382,.T.);
#2861=ADVANCED_FACE('',(#501,#321,#322,#323,#324,#325),#383,.F.);
#2862=ADVANCED_FACE('',(#502,#326,#327,#328,#329,#330),#384,.T.);
#2863=ADVANCED_FACE('',(#503),#385,.F.);
#2864=ADVANCED_FACE('',(#504),#386,.F.);
#2865=ADVANCED_FACE('',(#505),#387,.F.);
#2866=ADVANCED_FACE('',(#506),#388,.F.);
#2867=ADVANCED_FACE('',(#507),#389,.F.);
#2868=ADVANCED_FACE('',(#508),#390,.F.);
#2869=ADVANCED_FACE('',(#509),#391,.F.);
#2870=ADVANCED_FACE('',(#510),#392,.F.);
#2962=CLOSED_SHELL('',(#2834,#2835,#2836,#2837,#2838,#2839,#2840,#2841,
#2842,#2843,#2844,#2845,#2846,#2847,#2848,#2849,#2850,#2851,#2852,#2853,
#2854,#2855,#2856,#2857,#2858,#2859,#2860,#2861,#2862,#2863,#2864,#2865,
#2866,#2867,#2868,#2869,#2870));
#3108=AXIS2_PLACEMENT_3D('',#4430,#3555,#3556);
#3109=AXIS2_PLACEMENT_3D('',#4431,#3557,#3558);
#3110=AXIS2_PLACEMENT_3D('',#4433,#3559,#3560);
#3111=AXIS2_PLACEMENT_3D('',#4436,#3562,#3563);
#3112=AXIS2_PLACEMENT_3D('',#4437,#3564,#3565);
#3113=AXIS2_PLACEMENT_3D('',#4439,#3566,#3567);
#3114=AXIS2_PLACEMENT_3D('',#4442,#3569,#3570);
#3115=AXIS2_PLACEMENT_3D('',#4443,#3571,#3572);
#3116=AXIS2_PLACEMENT_3D('',#4445,#3573,#3574);
#3117=AXIS2_PLACEMENT_3D('',#4448,#3576,#3577);
#3118=AXIS2_PLACEMENT_3D('',#4449,#3578,#3579);
#3119=AXIS2_PLACEMENT_3D('',#4451,#3580,#3581);
#3120=AXIS2_PLACEMENT_3D('',#4454,#3583,#3584);
#3121=AXIS2_PLACEMENT_3D('',#4455,#3585,#3586);
#3122=AXIS2_PLACEMENT_3D('',#4457,#3587,#3588);
#3123=AXIS2_PLACEMENT_3D('',#4460,#3590,#3591);
#3124=AXIS2_PLACEMENT_3D('',#4461,#3592,#3593);
#3125=AXIS2_PLACEMENT_3D('',#4470,#3598,#3599);
#3126=AXIS2_PLACEMENT_3D('',#4476,#3603,#3604);
#3127=AXIS2_PLACEMENT_3D('',#4482,#3608,#3609);
#3128=AXIS2_PLACEMENT_3D('',#4485,#3612,#3613);
#3129=AXIS2_PLACEMENT_3D('',#4494,#3618,#3619);
#3130=AXIS2_PLACEMENT_3D('',#4500,#3623,#3624);
#3131=AXIS2_PLACEMENT_3D('',#4506,#3628,#3629);
#3132=AXIS2_PLACEMENT_3D('',#4509,#3632,#3633);
#3133=AXIS2_PLACEMENT_3D('',#4518,#3638,#3639);
#3134=AXIS2_PLACEMENT_3D('',#4524,#3643,#3644);
#3135=AXIS2_PLACEMENT_3D('',#4530,#3648,#3649);
#3136=AXIS2_PLACEMENT_3D('',#4533,#3652,#3653);
#3137=AXIS2_PLACEMENT_3D('',#4542,#3658,#3659);
#3138=AXIS2_PLACEMENT_3D('',#4548,#3663,#3664);
#3139=AXIS2_PLACEMENT_3D('',#4554,#3668,#3669);
#3140=AXIS2_PLACEMENT_3D('',#4557,#3672,#3673);
#3141=AXIS2_PLACEMENT_3D('',#4570,#3680,#3681);
#3142=AXIS2_PLACEMENT_3D('',#4583,#3688,#3689);
#3143=AXIS2_PLACEMENT_3D('',#4586,#3692,#3693);
#3144=AXIS2_PLACEMENT_3D('',#4604,#3703,#3704);
#3145=AXIS2_PLACEMENT_3D('',#4622,#3714,#3715);
#3146=AXIS2_PLACEMENT_3D('',#4625,#3718,#3719);
#3147=AXIS2_PLACEMENT_3D('',#4626,#3720,#3721);
#3148=AXIS2_PLACEMENT_3D('',#4627,#3722,#3723);
#3149=AXIS2_PLACEMENT_3D('',#4630,#3726,#3727);
#3150=AXIS2_PLACEMENT_3D('',#4632,#3729,#3730);
#3151=AXIS2_PLACEMENT_3D('',#4634,#3732,#3733);
#3152=AXIS2_PLACEMENT_3D('',#4635,#3734,#3735);
#3153=AXIS2_PLACEMENT_3D('',#4638,#3738,#3739);
#3154=AXIS2_PLACEMENT_3D('',#4640,#3741,#3742);
#3155=AXIS2_PLACEMENT_3D('',#4642,#3744,#3745);
#3555=DIRECTION('axis',(0.,0.,1.));
#3556=DIRECTION('refdir',(1.,0.,0.));
#3557=DIRECTION('center_axis',(0.,1.,0.));
#3558=DIRECTION('ref_axis',(0.,0.,1.));
#3559=DIRECTION('center_axis',(0.,1.,0.));
#3560=DIRECTION('ref_axis',(0.,0.,1.));
#3561=DIRECTION('',(0.,1.,0.));
#3562=DIRECTION('center_axis',(0.,1.,0.));
#3563=DIRECTION('ref_axis',(0.,0.,1.));
#3564=DIRECTION('center_axis',(0.,1.,0.));
#3565=DIRECTION('ref_axis',(0.,0.,1.));
#3566=DIRECTION('center_axis',(0.,1.,0.));
#3567=DIRECTION('ref_axis',(0.,0.,1.));
#3568=DIRECTION('',(0.,1.,0.));
#3569=DIRECTION('center_axis',(0.,1.,0.));
#3570=DIRECTION('ref_axis',(0.,0.,1.));
#3571=DIRECTION('center_axis',(0.,1.,0.));
#3572=DIRECTION('ref_axis',(0.,0.,1.));
#3573=DIRECTION('center_axis',(0.,1.,0.));
#3574=DIRECTION('ref_axis',(0.,0.,1.));
#3575=DIRECTION('',(0.,1.,0.));
#3576=DIRECTION('center_axis',(0.,1.,0.));
#3577=DIRECTION('ref_axis',(0.,0.,1.));
#3578=DIRECTION('center_axis',(0.,1.,0.));
#3579=DIRECTION('ref_axis',(0.,0.,1.));
#3580=DIRECTION('center_axis',(0.,1.,0.));
#3581=DIRECTION('ref_axis',(0.,0.,1.));
#3582=DIRECTION('',(0.,1.,0.));
#3583=DIRECTION('center_axis',(0.,1.,0.));
#3584=DIRECTION('ref_axis',(0.,0.,1.));
#3585=DIRECTION('center_axis',(0.,1.,0.));
#3586=DIRECTION('ref_axis',(0.,0.,1.));
#3587=DIRECTION('center_axis',(0.,1.,0.));
#3588=DIRECTION('ref_axis',(0.,0.,1.));
#3589=DIRECTION('',(0.,1.,0.));
#3590=DIRECTION('center_axis',(0.,1.,0.));
#3591=DIRECTION('ref_axis',(0.,0.,1.));
#3592=DIRECTION('center_axis',(0.,-1.,0.));
#3593=DIRECTION('ref_axis',(0.,0.,-1.));
#3594=DIRECTION('',(0.,0.,1.));
#3595=DIRECTION('',(1.,0.,0.));
#3596=DIRECTION('',(0.,0.,1.));
#3597=DIRECTION('',(1.,0.,0.));
#3598=DIRECTION('center_axis',(1.,0.,0.));
#3599=DIRECTION('ref_axis',(0.,0.,-1.));
#3600=DIRECTION('',(0.,1.,0.));
#3601=DIRECTION('',(0.,0.,1.));
#3602=DIRECTION('',(0.,1.,0.));
#3603=DIRECTION('center_axis',(0.,1.,0.));
#3604=DIRECTION('ref_axis',(0.,0.,1.));
#3605=DIRECTION('',(-1.,0.,0.));
#3606=DIRECTION('',(0.,0.,1.));
#3607=DIRECTION('',(-1.,0.,0.));
#3608=DIRECTION('center_axis',(-1.,0.,0.));
#3609=DIRECTION('ref_axis',(0.,0.,1.));
#3610=DIRECTION('',(0.,-1.,0.));
#3611=DIRECTION('',(0.,-1.,0.));
#3612=DIRECTION('center_axis',(0.,-1.,0.));
#3613=DIRECTION('ref_axis',(0.,0.,-1.));
#3614=DIRECTION('',(0.,0.,1.));
#3615=DIRECTION('',(1.,0.,0.));
#3616=DIRECTION('',(0.,0.,1.));
#3617=DIRECTION('',(1.,0.,0.));
#3618=DIRECTION('center_axis',(1.,0.,0.));
#3619=DIRECTION('ref_axis',(0.,0.,-1.));
#3620=DIRECTION('',(0.,1.,0.));
#3621=DIRECTION('',(0.,0.,1.));
#3622=DIRECTION('',(0.,1.,0.));
#3623=DIRECTION('center_axis',(0.,1.,0.));
#3624=DIRECTION('ref_axis',(0.,0.,1.));
#3625=DIRECTION('',(-1.,0.,0.));
#3626=DIRECTION('',(0.,0.,1.));
#3627=DIRECTION('',(-1.,0.,0.));
#3628=DIRECTION('center_axis',(-1.,0.,0.));
#3629=DIRECTION('ref_axis',(0.,0.,1.));
#3630=DIRECTION('',(0.,-1.,0.));
#3631=DIRECTION('',(0.,-1.,0.));
#3632=DIRECTION('center_axis',(0.,-1.,0.));
#3633=DIRECTION('ref_axis',(0.,0.,-1.));
#3634=DIRECTION('',(0.,0.,1.));
#3635=DIRECTION('',(1.,0.,0.));
#3636=DIRECTION('',(0.,0.,1.));
#3637=DIRECTION('',(1.,0.,0.));
#3638=DIRECTION('center_axis',(1.,0.,0.));
#3639=DIRECTION('ref_axis',(0.,0.,-1.));
#3640=DIRECTION('',(0.,1.,0.));
#3641=DIRECTION('',(0.,0.,1.));
#3642=DIRECTION('',(0.,1.,0.));
#3643=DIRECTION('center_axis',(0.,1.,0.));
#3644=DIRECTION('ref_axis',(0.,0.,1.));
#3645=DIRECTION('',(-1.,0.,0.));
#3646=DIRECTION('',(0.,0.,1.));
#3647=DIRECTION('',(-1.,0.,0.));
#3648=DIRECTION('center_axis',(-1.,0.,0.));
#3649=DIRECTION('ref_axis',(0.,0.,1.));
#3650=DIRECTION('',(0.,-1.,0.));
#3651=DIRECTION('',(0.,-1.,0.));
#3652=DIRECTION('center_axis',(0.,-1.,0.));
#3653=DIRECTION('ref_axis',(0.,0.,-1.));
#3654=DIRECTION('',(0.,0.,1.));
#3655=DIRECTION('',(1.,0.,0.));
#3656=DIRECTION('',(0.,0.,1.));
#3657=DIRECTION('',(1.,0.,0.));
#3658=DIRECTION('center_axis',(1.,0.,0.));
#3659=DIRECTION('ref_axis',(0.,0.,-1.));
#3660=DIRECTION('',(0.,1.,0.));
#3661=DIRECTION('',(0.,0.,1.));
#3662=DIRECTION('',(0.,1.,0.));
#3663=DIRECTION('center_axis',(0.,1.,0.));
#3664=DIRECTION('ref_axis',(0.,0.,1.));
#3665=DIRECTION('',(-1.,0.,0.));
#3666=DIRECTION('',(0.,0.,1.));
#3667=DIRECTION('',(-1.,0.,0.));
#3668=DIRECTION('center_axis',(-1.,0.,0.));
#3669=DIRECTION('ref_axis',(0.,0.,1.));
#3670=DIRECTION('',(0.,-1.,0.));
#3671=DIRECTION('',(0.,-1.,0.));
#3672=DIRECTION('center_axis',(1.,0.,0.));
#3673=DIRECTION('ref_axis',(0.,0.,-1.));
#3674=DIRECTION('',(0.,-1.,0.));
#3675=DIRECTION('',(0.,0.,1.));
#3676=DIRECTION('',(0.,1.,0.));
#3677=DIRECTION('',(0.,0.,1.));
#3678=DIRECTION('',(0.,-1.,0.));
#3679=DIRECTION('',(0.,0.,-1.));
#3680=DIRECTION('center_axis',(-1.,0.,0.));
#3681=DIRECTION('ref_axis',(0.,0.,1.));
#3682=DIRECTION('',(0.,1.,0.));
#3683=DIRECTION('',(0.,0.,-1.));
#3684=DIRECTION('',(0.,1.,0.));
#3685=DIRECTION('',(0.,0.,-1.));
#3686=DIRECTION('',(0.,1.,0.));
#3687=DIRECTION('',(0.,0.,-1.));
#3688=DIRECTION('center_axis',(0.,-1.,0.));
#3689=DIRECTION('ref_axis',(0.,0.,-1.));
#3690=DIRECTION('',(-1.,0.,0.));
#3691=DIRECTION('',(-1.,0.,0.));
#3692=DIRECTION('center_axis',(0.,0.,-1.));
#3693=DIRECTION('ref_axis',(-1.,0.,0.));
#3694=DIRECTION('',(-1.,0.,0.));
#3695=DIRECTION('',(1.,0.,0.));
#3696=DIRECTION('',(0.,-1.,0.));
#3697=DIRECTION('',(-1.,0.,0.));
#3698=DIRECTION('',(0.,1.,0.));
#3699=DIRECTION('',(1.,0.,0.));
#3700=DIRECTION('',(0.,-1.,0.));
#3701=DIRECTION('',(-1.,0.,0.));
#3702=DIRECTION('',(0.,1.,0.));
#3703=DIRECTION('center_axis',(0.,0.,-1.));
#3704=DIRECTION('ref_axis',(-1.,0.,0.));
#3705=DIRECTION('',(1.,0.,0.));
#3706=DIRECTION('',(0.,-1.,0.));
#3707=DIRECTION('',(1.,0.,0.));
#3708=DIRECTION('',(0.,1.,0.));
#3709=DIRECTION('',(-1.,0.,0.));
#3710=DIRECTION('',(0.,-1.,0.));
#3711=DIRECTION('',(1.,0.,0.));
#3712=DIRECTION('',(0.,1.,0.));
#3713=DIRECTION('',(-1.,0.,0.));
#3714=DIRECTION('center_axis',(0.,0.,1.));
#3715=DIRECTION('ref_axis',(1.,0.,0.));
#3716=DIRECTION('',(1.,0.,0.));
#3717=DIRECTION('',(1.,0.,0.));
#3718=DIRECTION('center_axis',(0.,1.,0.));
#3719=DIRECTION('ref_axis',(-1.,0.,0.));
#3720=DIRECTION('center_axis',(0.,1.,0.));
#3721=DIRECTION('ref_axis',(-1.,0.,0.));
#3722=DIRECTION('center_axis',(-1.,0.,0.));
#3723=DIRECTION('ref_axis',(0.,0.,1.));
#3724=DIRECTION('',(0.,0.,1.));
#3725=DIRECTION('',(0.,0.,1.));
#3726=DIRECTION('center_axis',(0.,1.,0.));
#3727=DIRECTION('ref_axis',(0.,0.,1.));
#3728=DIRECTION('',(0.,0.,1.));
#3729=DIRECTION('center_axis',(1.,0.,0.));
#3730=DIRECTION('ref_axis',(0.,0.,-1.));
#3731=DIRECTION('',(0.,0.,1.));
#3732=DIRECTION('center_axis',(0.,-1.,0.));
#3733=DIRECTION('ref_axis',(0.,0.,-1.));
#3734=DIRECTION('center_axis',(-1.,0.,0.));
#3735=DIRECTION('ref_axis',(0.,0.,1.));
#3736=DIRECTION('',(0.,0.,1.));
#3737=DIRECTION('',(0.,0.,1.));
#3738=DIRECTION('center_axis',(0.,1.,0.));
#3739=DIRECTION('ref_axis',(0.,0.,1.));
#3740=DIRECTION('',(0.,0.,1.));
#3741=DIRECTION('center_axis',(1.,0.,0.));
#3742=DIRECTION('ref_axis',(0.,0.,-1.));
#3743=DIRECTION('',(0.,0.,1.));
#3744=DIRECTION('center_axis',(0.,-1.,0.));
#3745=DIRECTION('ref_axis',(0.,0.,-1.));
#4430=CARTESIAN_POINT('',(0.,0.,0.));
#4431=CARTESIAN_POINT('Origin',(53.3333333333333,-20.,162.5));
#4432=CARTESIAN_POINT('',(53.3333333333333,-25.,159.85));
#4433=CARTESIAN_POINT('Origin',(53.3333333333333,-25.,162.5));
#4434=CARTESIAN_POINT('',(53.3333333333333,-20.,159.85));
#4435=CARTESIAN_POINT('',(53.3333333333333,-20.,159.85));
#4436=CARTESIAN_POINT('Origin',(53.3333333333333,-20.,162.5));
#4437=CARTESIAN_POINT('Origin',(136.666666666667,-20.,162.5));
#4438=CARTESIAN_POINT('',(136.666666666667,-25.,159.85));
#4439=CARTESIAN_POINT('Origin',(136.666666666667,-25.,162.5));
#4440=CARTESIAN_POINT('',(136.666666666667,-20.,159.85));
#4441=CARTESIAN_POINT('',(136.666666666667,-20.,159.85));
#4442=CARTESIAN_POINT('Origin',(136.666666666667,-20.,162.5));
#4443=CARTESIAN_POINT('Origin',(220.,-20.,162.5));
#4444=CARTESIAN_POINT('',(220.,-25.,159.85));
#4445=CARTESIAN_POINT('Origin',(220.,-25.,162.5));
#4446=CARTESIAN_POINT('',(220.,-20.,159.85));
#4447=CARTESIAN_POINT('',(220.,-20.,159.85));
#4448=CARTESIAN_POINT('Origin',(220.,-20.,162.5));
#4449=CARTESIAN_POINT('Origin',(303.333333333333,-20.,162.5));
#4450=CARTESIAN_POINT('',(303.333333333333,-25.,159.85));
#4451=CARTESIAN_POINT('Origin',(303.333333333333,-25.,162.5));
#4452=CARTESIAN_POINT('',(303.333333333333,-20.,159.85));
#4453=CARTESIAN_POINT('',(303.333333333333,-20.,159.85));
#4454=CARTESIAN_POINT('Origin',(303.333333333333,-20.,162.5));
#4455=CARTESIAN_POINT('Origin',(386.666666666667,-20.,162.5));
#4456=CARTESIAN_POINT('',(386.666666666667,-25.,159.85));
#4457=CARTESIAN_POINT('Origin',(386.666666666667,-25.,162.5));
#4458=CARTESIAN_POINT('',(386.666666666667,-20.,159.85));
#4459=CARTESIAN_POINT('',(386.666666666667,-20.,159.85));
#4460=CARTESIAN_POINT('Origin',(386.666666666667,-20.,162.5));
#4461=CARTESIAN_POINT('Origin',(435.,-8.66025403784439,139.999));
#4462=CARTESIAN_POINT('',(435.,-8.66025403784439,140.));
#4463=CARTESIAN_POINT('',(435.,-8.66025403784439,145.));
#4464=CARTESIAN_POINT('',(435.,-8.66025403784439,139.999));
#4465=CARTESIAN_POINT('',(445.,-8.66025403784439,145.));
#4466=CARTESIAN_POINT('',(435.,-8.66025403784439,145.));
#4467=CARTESIAN_POINT('',(445.,-8.66025403784439,140.));
#4468=CARTESIAN_POINT('',(445.,-8.66025403784439,139.999));
#4469=CARTESIAN_POINT('',(435.,-8.66025403784439,140.));
#4470=CARTESIAN_POINT('Origin',(445.,8.66025403784439,139.999));
#4471=CARTESIAN_POINT('',(445.,8.66025403784439,145.));
#4472=CARTESIAN_POINT('',(445.,8.66025403784439,145.));
#4473=CARTESIAN_POINT('',(445.,8.66025403784439,140.));
#4474=CARTESIAN_POINT('',(445.,8.66025403784439,139.999));
#4475=CARTESIAN_POINT('',(445.,8.66025403784439,140.));
#4476=CARTESIAN_POINT('Origin',(435.,8.66025403784439,139.999));
#4477=CARTESIAN_POINT('',(435.,8.66025403784439,145.));
#4478=CARTESIAN_POINT('',(435.,8.66025403784439,145.));
#4479=CARTESIAN_POINT('',(435.,8.66025403784439,140.));
#4480=CARTESIAN_POINT('',(435.,8.66025403784439,139.999));
#4481=CARTESIAN_POINT('',(435.,8.66025403784439,140.));
#4482=CARTESIAN_POINT('Origin',(435.,8.66025403784439,139.999));
#4483=CARTESIAN_POINT('',(435.,8.66025403784439,145.));
#4484=CARTESIAN_POINT('',(435.,8.66025403784439,140.));
#4485=CARTESIAN_POINT('Origin',(347.,-8.66025403784439,139.999));
#4486=CARTESIAN_POINT('',(347.,-8.66025403784439,140.));
#4487=CARTESIAN_POINT('',(347.,-8.66025403784439,145.));
#4488=CARTESIAN_POINT('',(347.,-8.66025403784439,139.999));
#4489=CARTESIAN_POINT('',(357.,-8.66025403784439,145.));
#4490=CARTESIAN_POINT('',(347.,-8.66025403784439,145.));
#4491=CARTESIAN_POINT('',(357.,-8.66025403784439,140.));
#4492=CARTESIAN_POINT('',(357.,-8.66025403784439,139.999));
#4493=CARTESIAN_POINT('',(347.,-8.66025403784439,140.));
#4494=CARTESIAN_POINT('Origin',(357.,8.66025403784439,139.999));
#4495=CARTESIAN_POINT('',(357.,8.66025403784439,145.));
#4496=CARTESIAN_POINT('',(357.,8.66025403784439,145.));
#4497=CARTESIAN_POINT('',(357.,8.66025403784439,140.));
#4498=CARTESIAN_POINT('',(357.,8.66025403784439,139.999));
#4499=CARTESIAN_POINT('',(357.,8.66025403784439,140.));
#4500=CARTESIAN_POINT('Origin',(347.,8.66025403784439,139.999));
#4501=CARTESIAN_POINT('',(347.,8.66025403784439,145.));
#4502=CARTESIAN_POINT('',(347.,8.66025403784439,145.));
#4503=CARTESIAN_POINT('',(347.,8.66025403784439,140.));
#4504=CARTESIAN_POINT('',(347.,8.66025403784439,139.999));
#4505=CARTESIAN_POINT('',(347.,8.66025403784439,140.));
#4506=CARTESIAN_POINT('Origin',(347.,8.66025403784439,139.999));
#4507=CARTESIAN_POINT('',(347.,8.66025403784439,145.));
#4508=CARTESIAN_POINT('',(347.,8.66025403784439,140.));
#4509=CARTESIAN_POINT('Origin',(259.,-8.66025403784439,139.999));
#4510=CARTESIAN_POINT('',(259.,-8.66025403784439,140.));
#4511=CARTESIAN_POINT('',(259.,-8.66025403784439,145.));
#4512=CARTESIAN_POINT('',(259.,-8.66025403784439,139.999));
#4513=CARTESIAN_POINT('',(269.,-8.66025403784439,145.));
#4514=CARTESIAN_POINT('',(259.,-8.66025403784439,145.));
#4515=CARTESIAN_POINT('',(269.,-8.66025403784439,140.));
#4516=CARTESIAN_POINT('',(269.,-8.66025403784439,139.999));
#4517=CARTESIAN_POINT('',(259.,-8.66025403784439,140.));
#4518=CARTESIAN_POINT('Origin',(269.,8.66025403784439,139.999));
#4519=CARTESIAN_POINT('',(269.,8.66025403784439,145.));
#4520=CARTESIAN_POINT('',(269.,8.66025403784439,145.));
#4521=CARTESIAN_POINT('',(269.,8.66025403784439,140.));
#4522=CARTESIAN_POINT('',(269.,8.66025403784439,139.999));
#4523=CARTESIAN_POINT('',(269.,8.66025403784439,140.));
#4524=CARTESIAN_POINT('Origin',(259.,8.66025403784439,139.999));
#4525=CARTESIAN_POINT('',(259.,8.66025403784439,145.));
#4526=CARTESIAN_POINT('',(259.,8.66025403784439,145.));
#4527=CARTESIAN_POINT('',(259.,8.66025403784439,140.));
#4528=CARTESIAN_POINT('',(259.,8.66025403784439,139.999));
#4529=CARTESIAN_POINT('',(259.,8.66025403784439,140.));
#4530=CARTESIAN_POINT('Origin',(259.,8.66025403784439,139.999));
#4531=CARTESIAN_POINT('',(259.,8.66025403784439,145.));
#4532=CARTESIAN_POINT('',(259.,8.66025403784439,140.));
#4533=CARTESIAN_POINT('Origin',(171.,-8.66025403784439,139.999));
#4534=CARTESIAN_POINT('',(171.,-8.66025403784439,140.));
#4535=CARTESIAN_POINT('',(171.,-8.66025403784439,145.));
#4536=CARTESIAN_POINT('',(171.,-8.66025403784439,139.999));
#4537=CARTESIAN_POINT('',(181.,-8.66025403784439,145.));
#4538=CARTESIAN_POINT('',(171.,-8.66025403784439,145.));
#4539=CARTESIAN_POINT('',(181.,-8.66025403784439,140.));
#4540=CARTESIAN_POINT('',(181.,-8.66025403784439,139.999));
#4541=CARTESIAN_POINT('',(171.,-8.66025403784439,140.));
#4542=CARTESIAN_POINT('Origin',(181.,8.66025403784439,139.999));
#4543=CARTESIAN_POINT('',(181.,8.66025403784439,145.));
#4544=CARTESIAN_POINT('',(181.,8.66025403784439,145.));
#4545=CARTESIAN_POINT('',(181.,8.66025403784439,140.));
#4546=CARTESIAN_POINT('',(181.,8.66025403784439,139.999));
#4547=CARTESIAN_POINT('',(181.,8.66025403784439,140.));
#4548=CARTESIAN_POINT('Origin',(171.,8.66025403784439,139.999));
#4549=CARTESIAN_POINT('',(171.,8.66025403784439,145.));
#4550=CARTESIAN_POINT('',(171.,8.66025403784439,145.));
#4551=CARTESIAN_POINT('',(171.,8.66025403784439,140.));
#4552=CARTESIAN_POINT('',(171.,8.66025403784439,139.999));
#4553=CARTESIAN_POINT('',(171.,8.66025403784439,140.));
#4554=CARTESIAN_POINT('Origin',(171.,8.66025403784439,139.999));
#4555=CARTESIAN_POINT('',(171.,8.66025403784439,145.));
#4556=CARTESIAN_POINT('',(171.,8.66025403784439,140.));
#4557=CARTESIAN_POINT('Origin',(-30.,0.,145.));
#4558=CARTESIAN_POINT('',(-30.,20.,140.));
#4559=CARTESIAN_POINT('',(-30.,-25.,140.));
#4560=CARTESIAN_POINT('',(-30.,0.,140.));
#4561=CARTESIAN_POINT('',(-30.,-25.,180.));
#4562=CARTESIAN_POINT('',(-30.,-25.,140.));
#4563=CARTESIAN_POINT('',(-30.,-20.,180.));
#4564=CARTESIAN_POINT('',(-30.,-25.,180.));
#4565=CARTESIAN_POINT('',(-30.,-20.,145.));
#4566=CARTESIAN_POINT('',(-30.,-20.,140.));
#4567=CARTESIAN_POINT('',(-30.,20.,145.));
#4568=CARTESIAN_POINT('',(-30.,0.,145.));
#4569=CARTESIAN_POINT('',(-30.,20.,145.));
#4570=CARTESIAN_POINT('Origin',(470.,0.,145.));
#4571=CARTESIAN_POINT('',(470.,-25.,140.));
#4572=CARTESIAN_POINT('',(470.,20.,140.));
#4573=CARTESIAN_POINT('',(470.,0.,140.));
#4574=CARTESIAN_POINT('',(470.,20.,145.));
#4575=CARTESIAN_POINT('',(470.,20.,145.));
#4576=CARTESIAN_POINT('',(470.,-20.,145.));
#4577=CARTESIAN_POINT('',(470.,0.,145.));
#4578=CARTESIAN_POINT('',(470.,-20.,180.));
#4579=CARTESIAN_POINT('',(470.,-20.,180.));
#4580=CARTESIAN_POINT('',(470.,-25.,180.));
#4581=CARTESIAN_POINT('',(470.,-25.,180.));
#4582=CARTESIAN_POINT('',(470.,-25.,180.));
#4583=CARTESIAN_POINT('Origin',(0.,20.,145.));
#4584=CARTESIAN_POINT('',(0.,20.,140.));
#4585=CARTESIAN_POINT('',(0.,20.,145.));
#4586=CARTESIAN_POINT('Origin',(0.,0.,145.));
#4587=CARTESIAN_POINT('',(0.,-20.,145.));
#4588=CARTESIAN_POINT('',(83.,-8.66025403784439,145.));
#4589=CARTESIAN_POINT('',(93.,-8.66025403784439,145.));
#4590=CARTESIAN_POINT('',(83.,-8.66025403784439,145.));
#4591=CARTESIAN_POINT('',(83.,8.66025403784439,145.));
#4592=CARTESIAN_POINT('',(83.,8.66025403784439,145.));
#4593=CARTESIAN_POINT('',(93.,8.66025403784439,145.));
#4594=CARTESIAN_POINT('',(83.,8.66025403784439,145.));
#4595=CARTESIAN_POINT('',(93.,8.66025403784439,145.));
#4596=CARTESIAN_POINT('',(-5.,-8.66025403784439,145.));
#4597=CARTESIAN_POINT('',(5.,-8.66025403784439,145.));
#4598=CARTESIAN_POINT('',(-5.,-8.66025403784439,145.));
#4599=CARTESIAN_POINT('',(-5.,8.66025403784439,145.));
#4600=CARTESIAN_POINT('',(-5.,8.66025403784439,145.));
#4601=CARTESIAN_POINT('',(5.,8.66025403784439,145.));
#4602=CARTESIAN_POINT('',(-5.,8.66025403784439,145.));
#4603=CARTESIAN_POINT('',(5.,8.66025403784439,145.));
#4604=CARTESIAN_POINT('Origin',(0.,0.,140.));
#4605=CARTESIAN_POINT('',(-30.,-25.,140.));
#4606=CARTESIAN_POINT('',(83.,8.66025403784439,140.));
#4607=CARTESIAN_POINT('',(83.,-8.66025403784439,140.));
#4608=CARTESIAN_POINT('',(83.,8.66025403784439,140.));
#4609=CARTESIAN_POINT('',(93.,-8.66025403784439,140.));
#4610=CARTESIAN_POINT('',(83.,-8.66025403784439,140.));
#4611=CARTESIAN_POINT('',(93.,8.66025403784439,140.));
#4612=CARTESIAN_POINT('',(93.,8.66025403784439,140.));
#4613=CARTESIAN_POINT('',(83.,8.66025403784439,140.));
#4614=CARTESIAN_POINT('',(-5.,8.66025403784439,140.));
#4615=CARTESIAN_POINT('',(-5.,-8.66025403784439,140.));
#4616=CARTESIAN_POINT('',(-5.,8.66025403784439,140.));
#4617=CARTESIAN_POINT('',(5.,-8.66025403784439,140.));
#4618=CARTESIAN_POINT('',(-5.,-8.66025403784439,140.));
#4619=CARTESIAN_POINT('',(5.,8.66025403784439,140.));
#4620=CARTESIAN_POINT('',(5.,8.66025403784439,140.));
#4621=CARTESIAN_POINT('',(-5.,8.66025403784439,140.));
#4622=CARTESIAN_POINT('Origin',(-30.,-25.,180.));
#4623=CARTESIAN_POINT('',(-30.,-20.,180.));
#4624=CARTESIAN_POINT('',(-30.,-25.,180.));
#4625=CARTESIAN_POINT('Origin',(0.,-25.,0.));
#4626=CARTESIAN_POINT('Origin',(0.,-20.,0.));
#4627=CARTESIAN_POINT('Origin',(-5.,8.66025403784439,139.999));
#4628=CARTESIAN_POINT('',(-5.,8.66025403784439,139.999));
#4629=CARTESIAN_POINT('',(-5.,-8.66025403784439,139.999));
#4630=CARTESIAN_POINT('Origin',(-5.,8.66025403784439,139.999));
#4631=CARTESIAN_POINT('',(5.,8.66025403784439,139.999));
#4632=CARTESIAN_POINT('Origin',(5.,8.66025403784439,139.999));
#4633=CARTESIAN_POINT('',(5.,-8.66025403784439,139.999));
#4634=CARTESIAN_POINT('Origin',(-5.,-8.66025403784439,139.999));
#4635=CARTESIAN_POINT('Origin',(83.,8.66025403784439,139.999));
#4636=CARTESIAN_POINT('',(83.,8.66025403784439,139.999));
#4637=CARTESIAN_POINT('',(83.,-8.66025403784439,139.999));
#4638=CARTESIAN_POINT('Origin',(83.,8.66025403784439,139.999));
#4639=CARTESIAN_POINT('',(93.,8.66025403784439,139.999));
#4640=CARTESIAN_POINT('Origin',(93.,8.66025403784439,139.999));
#4641=CARTESIAN_POINT('',(93.,-8.66025403784439,139.999));
#4642=CARTESIAN_POINT('Origin',(83.,-8.66025403784439,139.999));
#5674=UNCERTAINTY_MEASURE_WITH_UNIT(LENGTH_MEASURE(0.01),#5690,
'DISTANCE_ACCURACY_VALUE',
'Maximum model space distance between geometric entities at asserted c
onnectivities');
#5680=UNCERTAINTY_MEASURE_WITH_UNIT(LENGTH_MEASURE(0.01),#5690,
'DISTANCE_ACCURACY_VALUE',
'Maximum model space distance between geometric entities at asserted c
onnectivities');
#5683=(
GEOMETRIC_REPRESENTATION_CONTEXT(3)
GLOBAL_UNCERTAINTY_ASSIGNED_CONTEXT((#5674))
GLOBAL_UNIT_ASSIGNED_CONTEXT((#5690,#5692,#5693))
REPRESENTATION_CONTEXT('','3D')
);
#5689=(
GEOMETRIC_REPRESENTATION_CONTEXT(3)
GLOBAL_UNCERTAINTY_ASSIGNED_CONTEXT((#5680))
GLOBAL_UNIT_ASSIGNED_CONTEXT((#5690,#5692,#5693))
REPRESENTATION_CONTEXT('','3D')
);
#5690=(
LENGTH_UNIT()
NAMED_UNIT(*)
SI_UNIT(.MILLI.,.METRE.)
);
#5692=(
NAMED_UNIT(*)
PLANE_ANGLE_UNIT()
SI_UNIT($,.RADIAN.)
);
#5693=(
NAMED_UNIT(*)
SI_UNIT($,.STERADIAN.)
SOLID_ANGLE_UNIT()
);
#5696=SHAPE_DEFINITION_REPRESENTATION(#5704,#5759);
#5704=PRODUCT_DEFINITION_SHAPE('',$,#5768);
#5759=SHAPE_REPRESENTATION('',(#3108),#5683);
#5765=PRODUCT_DEFINITION_CONTEXT('part definition',#5791,'design');
#5768=PRODUCT_DEFINITION('side rail','side rail',#5776,#5765);
#5776=PRODUCT_DEFINITION_FORMATION('',$,#5795);
#5791=APPLICATION_CONTEXT(
'Core Data for Automotive Mechanical Design Process');
#5792=PRODUCT_CONTEXT('part definition',#5791,'mechanical');
#5795=PRODUCT('side rail','side rail',$,(#5792));
#5803=PRESENTATION_STYLE_ASSIGNMENT((#5809));
#5809=SURFACE_STYLE_USAGE(.BOTH.,#5815);
#5815=SURFACE_SIDE_STYLE('',(#5821));
#5821=SURFACE_STYLE_FILL_AREA(#5827);
#5827=FILL_AREA_STYLE('Opaque(97,158,199)',(#5833));
#5833=FILL_AREA_STYLE_COLOUR('Opaque(97,158,199)',#5839);
#5839=COLOUR_RGB('Opaque(97,158,199)',0.380392156862745,0.619607843137255,
0.780392156862745);
ENDSEC;
END-ISO-10303-21;
